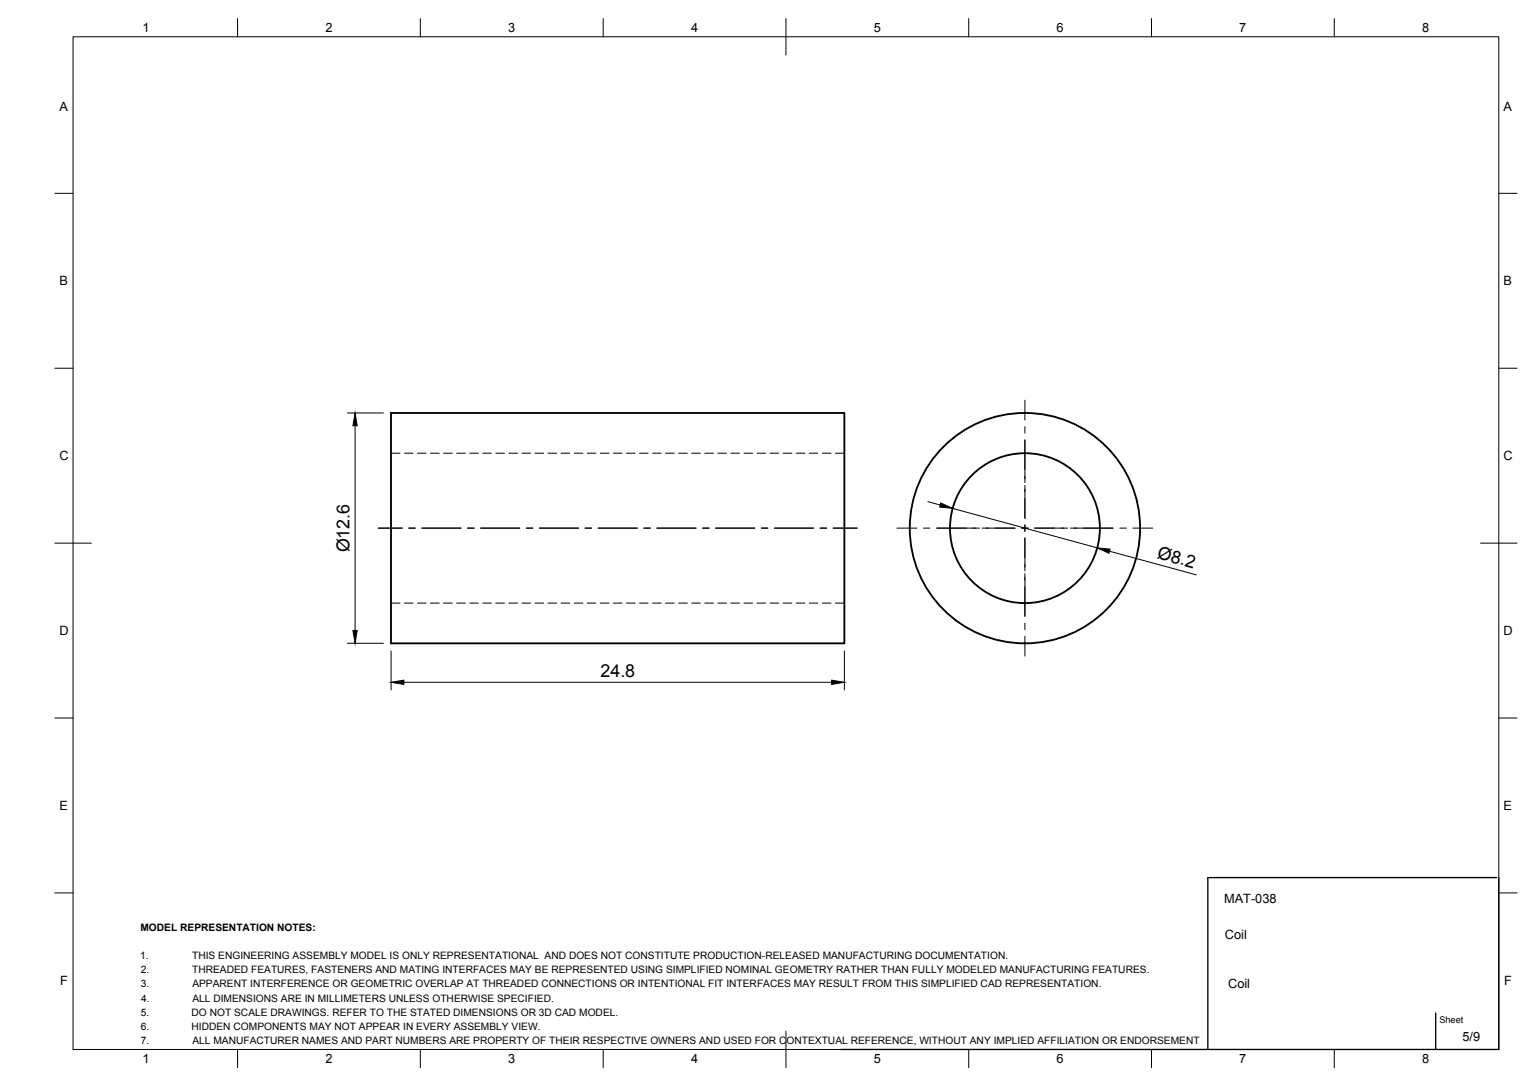
ISO-10303-21;
HEADER;
/* Generated by software containing ST-Developer
 * from STEP Tools, Inc. (www.steptools.com) 
 */

FILE_DESCRIPTION(
/* description */ ('STEP AP214'),
/* implementation_level */ '2;1');

FILE_NAME(
/* name */ 'Coil.step',
/* time_stamp */ '2026-11-14T21:32:33-08:00',
/* author */ (''),
/* organization */ (''),
/* preprocessor_version */ 'ST-DEVELOPER v20.2',
/* originating_system */ 'Autodesk Translation Framework v15.17.0.0',
/* authorisation */ '');

FILE_SCHEMA (('AUTOMOTIVE_DESIGN { 1 0 10303 214 3 1 1 }'));
ENDSEC;

DATA;
#10=MECHANICAL_DESIGN_GEOMETRIC_PRESENTATION_REPRESENTATION('',(#179),#10551);
#161=SHAPE_REPRESENTATION_RELATIONSHIP('SRR','None',#10588,#170);
#170=ADVANCED_BREP_SHAPE_REPRESENTATION('',(#189),#10544);
#179=STYLED_ITEM('',(#10642),#189);
#189=MANIFOLD_SOLID_BREP('Body1',#3428);
#208=FACE_BOUND('',#577,.T.);
#209=FACE_BOUND('',#579,.T.);
#255=PLANE('',#3631);
#256=PLANE('',#3632);
#343=FACE_OUTER_BOUND('',#574,.T.);
#344=FACE_OUTER_BOUND('',#575,.T.);
#345=FACE_OUTER_BOUND('',#576,.T.);
#346=FACE_OUTER_BOUND('',#578,.T.);
#574=EDGE_LOOP('',(#2440,#2441,#2442,#2443));
#575=EDGE_LOOP('',(#2444,#2445,#2446,#2447));
#576=EDGE_LOOP('',(#2448));
#577=EDGE_LOOP('',(#2449));
#578=EDGE_LOOP('',(#2450));
#579=EDGE_LOOP('',(#2451));
#851=LINE('',#5500,#1048);
#852=LINE('',#5506,#1049);
#1048=VECTOR('',#4308,6.3);
#1049=VECTOR('',#4315,4.1);
#1191=CIRCLE('',#3626,6.3);
#1192=CIRCLE('',#3627,6.3);
#1193=CIRCLE('',#3629,4.1);
#1194=CIRCLE('',#3630,4.1);
#1505=VERTEX_POINT('',#5497);
#1506=VERTEX_POINT('',#5499);
#1507=VERTEX_POINT('',#5503);
#1508=VERTEX_POINT('',#5505);
#1833=EDGE_CURVE('',#1505,#1505,#1191,.T.);
#1834=EDGE_CURVE('',#1505,#1506,#851,.T.);
#1835=EDGE_CURVE('',#1506,#1506,#1192,.T.);
#1836=EDGE_CURVE('',#1507,#1507,#1193,.T.);
#1837=EDGE_CURVE('',#1507,#1508,#852,.T.);
#1838=EDGE_CURVE('',#1508,#1508,#1194,.T.);
#2440=ORIENTED_EDGE('',*,*,#1833,.F.);
#2441=ORIENTED_EDGE('',*,*,#1834,.T.);
#2442=ORIENTED_EDGE('',*,*,#1835,.T.);
#2443=ORIENTED_EDGE('',*,*,#1834,.F.);
#2444=ORIENTED_EDGE('',*,*,#1836,.F.);
#2445=ORIENTED_EDGE('',*,*,#1837,.T.);
#2446=ORIENTED_EDGE('',*,*,#1838,.T.);
#2447=ORIENTED_EDGE('',*,*,#1837,.F.);
#2448=ORIENTED_EDGE('',*,*,#1833,.T.);
#2449=ORIENTED_EDGE('',*,*,#1838,.F.);
#2450=ORIENTED_EDGE('',*,*,#1835,.F.);
#2451=ORIENTED_EDGE('',*,*,#1836,.T.);
#3168=CYLINDRICAL_SURFACE('',#3625,6.3);
#3169=CYLINDRICAL_SURFACE('',#3628,4.1);
#3255=ADVANCED_FACE('',(#343),#3168,.T.);
#3256=ADVANCED_FACE('',(#344),#3169,.F.);
#3257=ADVANCED_FACE('',(#345,#208),#255,.F.);
#3258=ADVANCED_FACE('',(#346,#209),#256,.F.);
#3428=CLOSED_SHELL('',(#3255,#3256,#3257,#3258));
#3624=AXIS2_PLACEMENT_3D('',#5495,#4302,#4303);
#3625=AXIS2_PLACEMENT_3D('',#5496,#4304,#4305);
#3626=AXIS2_PLACEMENT_3D('',#5498,#4306,#4307);
#3627=AXIS2_PLACEMENT_3D('',#5501,#4309,#4310);
#3628=AXIS2_PLACEMENT_3D('',#5502,#4311,#4312);
#3629=AXIS2_PLACEMENT_3D('',#5504,#4313,#4314);
#3630=AXIS2_PLACEMENT_3D('',#5507,#4316,#4317);
#3631=AXIS2_PLACEMENT_3D('',#5508,#4318,#4319);
#3632=AXIS2_PLACEMENT_3D('',#5509,#4320,#4321);
#4302=DIRECTION('axis',(0.,0.,1.));
#4303=DIRECTION('refdir',(1.,0.,0.));
#4304=DIRECTION('center_axis',(-1.,0.,0.));
#4305=DIRECTION('ref_axis',(0.,0.,1.));
#4306=DIRECTION('center_axis',(-1.,0.,0.));
#4307=DIRECTION('ref_axis',(0.,0.,1.));
#4308=DIRECTION('',(1.,0.,0.));
#4309=DIRECTION('center_axis',(-1.,0.,0.));
#4310=DIRECTION('ref_axis',(0.,0.,1.));
#4311=DIRECTION('center_axis',(-1.,0.,0.));
#4312=DIRECTION('ref_axis',(0.,0.,1.));
#4313=DIRECTION('center_axis',(-1.,0.,0.));
#4314=DIRECTION('ref_axis',(0.,0.,1.));
#4315=DIRECTION('',(-1.,0.,0.));
#4316=DIRECTION('center_axis',(-1.,0.,0.));
#4317=DIRECTION('ref_axis',(0.,0.,1.));
#4318=DIRECTION('center_axis',(1.,0.,0.));
#4319=DIRECTION('ref_axis',(0.,0.,-1.));
#4320=DIRECTION('center_axis',(-1.,0.,0.));
#4321=DIRECTION('ref_axis',(0.,0.,1.));
#5495=CARTESIAN_POINT('',(0.,0.,0.));
#5496=CARTESIAN_POINT('Origin',(-12.4,0.,0.));
#5497=CARTESIAN_POINT('',(-12.4,-7.71527483462833E-16,-6.3));
#5498=CARTESIAN_POINT('Origin',(-12.4,0.,0.));
#5499=CARTESIAN_POINT('',(12.4,-7.71527483462833E-16,-6.3));
#5500=CARTESIAN_POINT('',(-12.4,-7.71527483462833E-16,-6.3));
#5501=CARTESIAN_POINT('Origin',(12.4,0.,0.));
#5502=CARTESIAN_POINT('Origin',(-12.4,0.,0.));
#5503=CARTESIAN_POINT('',(12.4,-5.02105187650415E-16,-4.1));
#5504=CARTESIAN_POINT('Origin',(12.4,0.,0.));
#5505=CARTESIAN_POINT('',(-12.4,-5.02105187650415E-16,-4.1));
#5506=CARTESIAN_POINT('',(-12.4,-5.02105187650415E-16,-4.1));
#5507=CARTESIAN_POINT('Origin',(-12.4,0.,0.));
#5508=CARTESIAN_POINT('Origin',(-12.4,6.3,0.));
#5509=CARTESIAN_POINT('Origin',(12.4,6.3,0.));
#10533=UNCERTAINTY_MEASURE_WITH_UNIT(LENGTH_MEASURE(0.01),#10552,
'DISTANCE_ACCURACY_VALUE',
'Maximum model space distance between geometric entities at asserted c
onnectivities');
#10540=UNCERTAINTY_MEASURE_WITH_UNIT(LENGTH_MEASURE(0.01),#10552,
'DISTANCE_ACCURACY_VALUE',
'Maximum model space distance between geometric entities at asserted c
onnectivities');
#10544=(
GEOMETRIC_REPRESENTATION_CONTEXT(3)
GLOBAL_UNCERTAINTY_ASSIGNED_CONTEXT((#10533))
GLOBAL_UNIT_ASSIGNED_CONTEXT((#10552,#10554,#10555))
REPRESENTATION_CONTEXT('','3D')
);
#10551=(
GEOMETRIC_REPRESENTATION_CONTEXT(3)
GLOBAL_UNCERTAINTY_ASSIGNED_CONTEXT((#10540))
GLOBAL_UNIT_ASSIGNED_CONTEXT((#10552,#10554,#10555))
REPRESENTATION_CONTEXT('','3D')
);
#10552=(
LENGTH_UNIT()
NAMED_UNIT(*)
SI_UNIT(.MILLI.,.METRE.)
);
#10554=(
NAMED_UNIT(*)
PLANE_ANGLE_UNIT()
SI_UNIT($,.RADIAN.)
);
#10555=(
NAMED_UNIT(*)
SI_UNIT($,.STERADIAN.)
SOLID_ANGLE_UNIT()
);
#10559=SHAPE_DEFINITION_REPRESENTATION(#10569,#10588);
#10569=PRODUCT_DEFINITION_SHAPE('',$,#10599);
#10588=SHAPE_REPRESENTATION('',(#3624),#10544);
#10595=PRODUCT_DEFINITION_CONTEXT('part definition',#10627,'design');
#10599=PRODUCT_DEFINITION('Coil','Coil',#10609,#10595);
#10609=PRODUCT_DEFINITION_FORMATION('',$,#10632);
#10627=APPLICATION_CONTEXT(
'Core Data for Automotive Mechanical Design Process');
#10628=PRODUCT_CONTEXT('part definition',#10627,'mechanical');
#10632=PRODUCT('Coil','Coil',$,(#10628));
#10642=PRESENTATION_STYLE_ASSIGNMENT((#10649));
#10649=SURFACE_STYLE_USAGE(.BOTH.,#10656);
#10656=SURFACE_SIDE_STYLE('',(#10663));
#10663=SURFACE_STYLE_FILL_AREA(#10670);
#10670=FILL_AREA_STYLE('Opaque(227,224,212)',(#10677));
#10677=FILL_AREA_STYLE_COLOUR('Opaque(227,224,212)',#10684);
#10684=COLOUR_RGB('Opaque(227,224,212)',0.890196078431372,0.87843137254902,
0.831372549019608);
ENDSEC;
END-ISO-10303-21;
